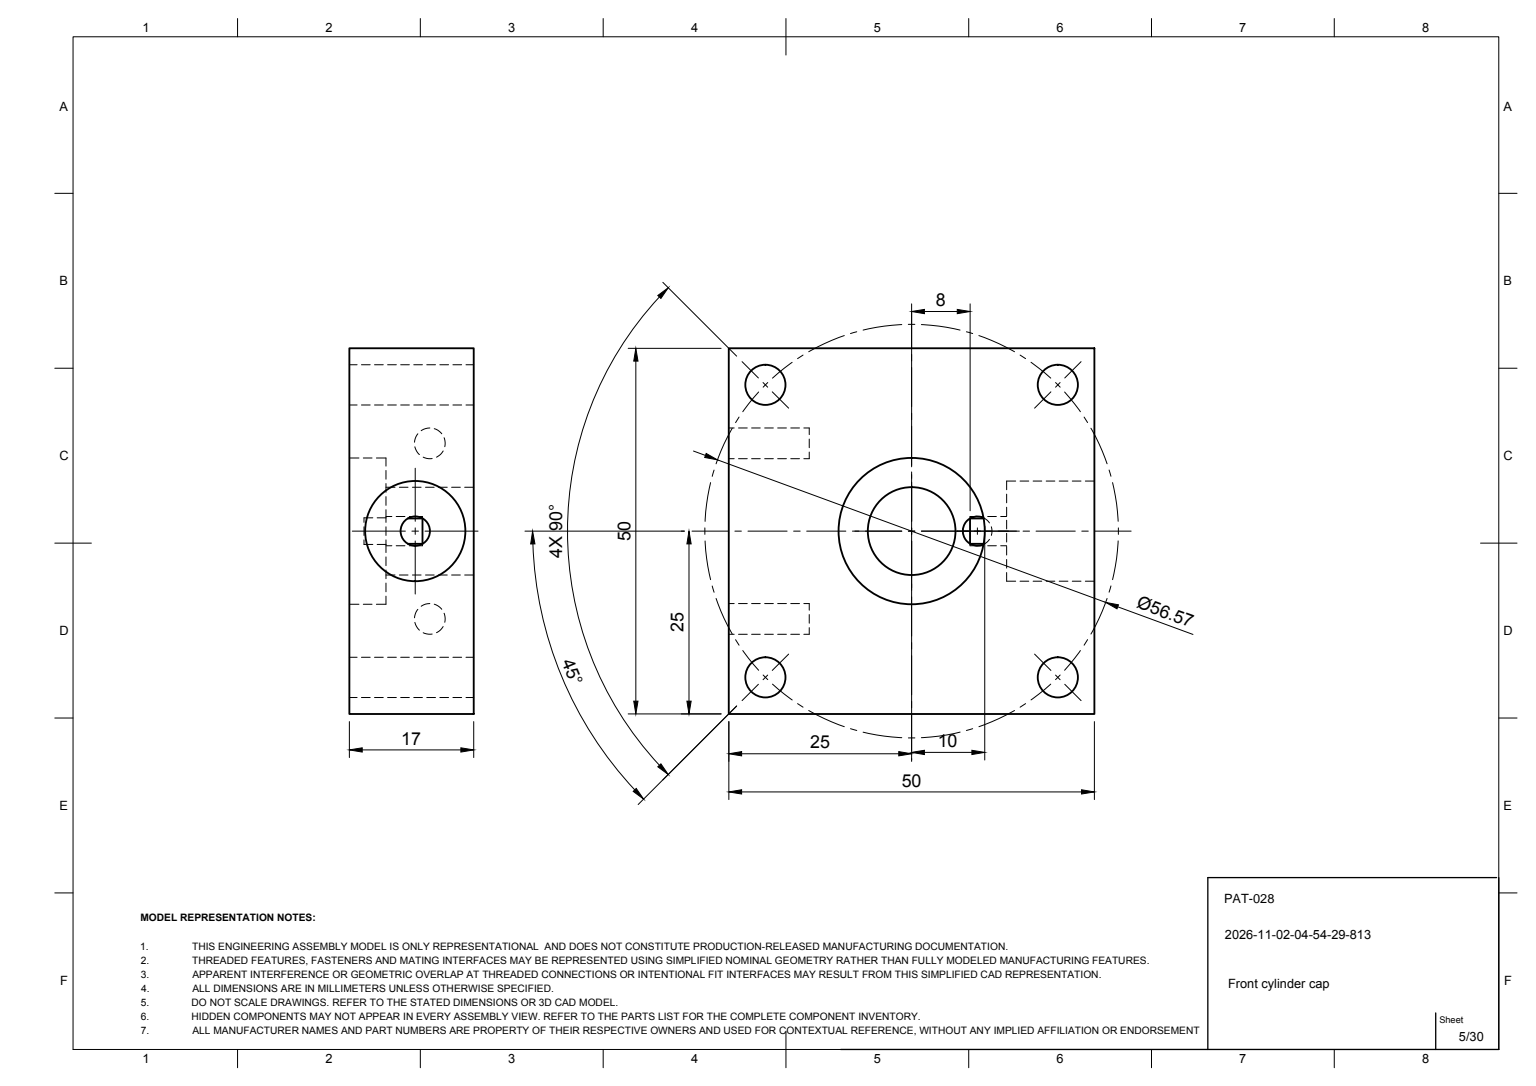
ISO-10303-21;
HEADER;
/* Generated by software containing ST-Developer
 * from STEP Tools, Inc. (www.steptools.com) 
 */

FILE_DESCRIPTION(
/* description */ ('Cylinder foot and clevis mount kit'),
/* implementation_level */ '2;1');

FILE_NAME(
/* name */ 'Front cylinder cap.step',
/* time_stamp */ '2026-10-27T20:10:43-07:00',
/* author */ (''),
/* organization */ (''),
/* preprocessor_version */ 'ST-DEVELOPER v20.2',
/* originating_system */ 'Autodesk Translation Framework v15.17.0.0',
/* authorisation */ '');

FILE_SCHEMA (('AUTOMOTIVE_DESIGN { 1 0 10303 214 3 1 1 }'));
ENDSEC;

DATA;
#10=MECHANICAL_DESIGN_GEOMETRIC_PRESENTATION_REPRESENTATION('',(#338),#9102);
#282=SHAPE_REPRESENTATION_RELATIONSHIP('SRR','None',#9229,#310);
#310=ADVANCED_BREP_SHAPE_REPRESENTATION('',(#366),#9072);
#338=STYLED_ITEM('',(#9446),#366);
#366=MANIFOLD_SOLID_BREP('Body1',#4924);
#392=FACE_BOUND('',#1021,.T.);
#393=FACE_BOUND('',#1028,.T.);
#394=FACE_BOUND('',#1030,.T.);
#395=FACE_BOUND('',#1031,.T.);
#396=FACE_BOUND('',#1032,.T.);
#397=FACE_BOUND('',#1033,.T.);
#398=FACE_BOUND('',#1034,.T.);
#399=FACE_BOUND('',#1037,.T.);
#400=FACE_BOUND('',#1038,.T.);
#401=FACE_BOUND('',#1039,.T.);
#402=FACE_BOUND('',#1040,.T.);
#403=FACE_BOUND('',#1041,.T.);
#404=FACE_BOUND('',#1044,.T.);
#405=FACE_BOUND('',#1046,.T.);
#406=FACE_BOUND('',#1047,.T.);
#495=ELLIPSE('',#5279,0.282842712474619,0.2);
#496=ELLIPSE('',#5280,0.282842712474619,0.2);
#497=ELLIPSE('',#5282,0.282842712474619,0.2);
#498=ELLIPSE('',#5283,0.282842712474619,0.2);
#499=ELLIPSE('',#5287,0.282842712474619,0.2);
#500=ELLIPSE('',#5289,0.282842712474619,0.2);
#501=ELLIPSE('',#5291,0.282842712474619,0.2);
#509=PLANE('',#5269);
#510=PLANE('',#5273);
#511=PLANE('',#5274);
#512=PLANE('',#5276);
#513=PLANE('',#5292);
#514=PLANE('',#5294);
#515=PLANE('',#5295);
#516=PLANE('',#5297);
#517=PLANE('',#5308);
#518=PLANE('',#5312);
#519=PLANE('',#5328);
#520=PLANE('',#5329);
#521=PLANE('',#5330);
#522=PLANE('',#5331);
#523=PLANE('',#5332);
#524=PLANE('',#5333);
#525=PLANE('',#5334);
#695=FACE_OUTER_BOUND('',#1001,.T.);
#696=FACE_OUTER_BOUND('',#1002,.T.);
#697=FACE_OUTER_BOUND('',#1003,.T.);
#698=FACE_OUTER_BOUND('',#1004,.T.);
#699=FACE_OUTER_BOUND('',#1005,.T.);
#700=FACE_OUTER_BOUND('',#1006,.T.);
#701=FACE_OUTER_BOUND('',#1007,.T.);
#702=FACE_OUTER_BOUND('',#1008,.T.);
#703=FACE_OUTER_BOUND('',#1009,.T.);
#704=FACE_OUTER_BOUND('',#1010,.T.);
#705=FACE_OUTER_BOUND('',#1011,.T.);
#706=FACE_OUTER_BOUND('',#1012,.T.);
#707=FACE_OUTER_BOUND('',#1013,.T.);
#708=FACE_OUTER_BOUND('',#1014,.T.);
#709=FACE_OUTER_BOUND('',#1015,.T.);
#710=FACE_OUTER_BOUND('',#1016,.T.);
#711=FACE_OUTER_BOUND('',#1017,.T.);
#712=FACE_OUTER_BOUND('',#1018,.T.);
#713=FACE_OUTER_BOUND('',#1019,.T.);
#714=FACE_OUTER_BOUND('',#1020,.T.);
#715=FACE_OUTER_BOUND('',#1022,.T.);
#716=FACE_OUTER_BOUND('',#1023,.T.);
#717=FACE_OUTER_BOUND('',#1024,.T.);
#718=FACE_OUTER_BOUND('',#1025,.T.);
#719=FACE_OUTER_BOUND('',#1026,.T.);
#720=FACE_OUTER_BOUND('',#1027,.T.);
#721=FACE_OUTER_BOUND('',#1029,.T.);
#722=FACE_OUTER_BOUND('',#1035,.T.);
#723=FACE_OUTER_BOUND('',#1036,.T.);
#724=FACE_OUTER_BOUND('',#1042,.T.);
#725=FACE_OUTER_BOUND('',#1043,.T.);
#726=FACE_OUTER_BOUND('',#1045,.T.);
#1001=EDGE_LOOP('',(#3315,#3316,#3317,#3318));
#1002=EDGE_LOOP('',(#3319));
#1003=EDGE_LOOP('',(#3320,#3321,#3322,#3323));
#1004=EDGE_LOOP('',(#3324));
#1005=EDGE_LOOP('',(#3325,#3326));
#1006=EDGE_LOOP('',(#3327,#3328));
#1007=EDGE_LOOP('',(#3329,#3330,#3331));
#1008=EDGE_LOOP('',(#3332,#3333,#3334,#3335,#3336,#3337,#3338,#3339,#3340,
#3341,#3342,#3343,#3344));
#1009=EDGE_LOOP('',(#3345,#3346,#3347));
#1010=EDGE_LOOP('',(#3348,#3349));
#1011=EDGE_LOOP('',(#3350,#3351));
#1012=EDGE_LOOP('',(#3352,#3353));
#1013=EDGE_LOOP('',(#3354,#3355));
#1014=EDGE_LOOP('',(#3356,#3357,#3358));
#1015=EDGE_LOOP('',(#3359,#3360,#3361,#3362,#3363,#3364,#3365,#3366,#3367));
#1016=EDGE_LOOP('',(#3368,#3369,#3370));
#1017=EDGE_LOOP('',(#3371,#3372,#3373,#3374,#3375,#3376,#3377,#3378));
#1018=EDGE_LOOP('',(#3379,#3380));
#1019=EDGE_LOOP('',(#3381,#3382,#3383,#3384));
#1020=EDGE_LOOP('',(#3385));
#1021=EDGE_LOOP('',(#3386));
#1022=EDGE_LOOP('',(#3387,#3388,#3389,#3390));
#1023=EDGE_LOOP('',(#3391,#3392,#3393,#3394));
#1024=EDGE_LOOP('',(#3395,#3396,#3397,#3398));
#1025=EDGE_LOOP('',(#3399,#3400,#3401,#3402));
#1026=EDGE_LOOP('',(#3403,#3404,#3405,#3406));
#1027=EDGE_LOOP('',(#3407,#3408,#3409,#3410));
#1028=EDGE_LOOP('',(#3411));
#1029=EDGE_LOOP('',(#3412,#3413,#3414,#3415));
#1030=EDGE_LOOP('',(#3416));
#1031=EDGE_LOOP('',(#3417));
#1032=EDGE_LOOP('',(#3418));
#1033=EDGE_LOOP('',(#3419));
#1034=EDGE_LOOP('',(#3420));
#1035=EDGE_LOOP('',(#3421,#3422,#3423,#3424));
#1036=EDGE_LOOP('',(#3425,#3426,#3427,#3428));
#1037=EDGE_LOOP('',(#3429));
#1038=EDGE_LOOP('',(#3430));
#1039=EDGE_LOOP('',(#3431));
#1040=EDGE_LOOP('',(#3432));
#1041=EDGE_LOOP('',(#3433));
#1042=EDGE_LOOP('',(#3434,#3435,#3436,#3437));
#1043=EDGE_LOOP('',(#3438,#3439,#3440,#3441));
#1044=EDGE_LOOP('',(#3442));
#1045=EDGE_LOOP('',(#3443,#3444,#3445,#3446));
#1046=EDGE_LOOP('',(#3447));
#1047=EDGE_LOOP('',(#3448));
#1410=LINE('',#7503,#1759);
#1411=LINE('',#7510,#1760);
#1412=LINE('',#7516,#1761);
#1413=LINE('',#7520,#1762);
#1414=LINE('',#7528,#1763);
#1415=LINE('',#7530,#1764);
#1416=LINE('',#7535,#1765);
#1417=LINE('',#7539,#1766);
#1418=LINE('',#7543,#1767);
#1419=LINE('',#7554,#1768);
#1420=LINE('',#7562,#1769);
#1421=LINE('',#7570,#1770);
#1422=LINE('',#7578,#1771);
#1423=LINE('',#7585,#1772);
#1424=LINE('',#7591,#1773);
#1425=LINE('',#7597,#1774);
#1426=LINE('',#7603,#1775);
#1427=LINE('',#7609,#1776);
#1428=LINE('',#7615,#1777);
#1429=LINE('',#7617,#1778);
#1430=LINE('',#7619,#1779);
#1431=LINE('',#7620,#1780);
#1432=LINE('',#7623,#1781);
#1433=LINE('',#7625,#1782);
#1434=LINE('',#7626,#1783);
#1435=LINE('',#7629,#1784);
#1436=LINE('',#7631,#1785);
#1437=LINE('',#7632,#1786);
#1438=LINE('',#7634,#1787);
#1439=LINE('',#7635,#1788);
#1759=VECTOR('',#5901,0.21);
#1760=VECTOR('',#5910,0.21);
#1761=VECTOR('',#5917,1.);
#1762=VECTOR('',#5922,1.);
#1763=VECTOR('',#5933,1.);
#1764=VECTOR('',#5934,1.);
#1765=VECTOR('',#5939,0.2);
#1766=VECTOR('',#5942,1.);
#1767=VECTOR('',#5945,1.);
#1768=VECTOR('',#5964,1.);
#1769=VECTOR('',#5977,0.2);
#1770=VECTOR('',#5988,1.);
#1771=VECTOR('',#5999,0.685);
#1772=VECTOR('',#6008,0.275);
#1773=VECTOR('',#6015,0.275);
#1774=VECTOR('',#6022,0.275);
#1775=VECTOR('',#6029,0.275);
#1776=VECTOR('',#6036,0.6);
#1777=VECTOR('',#6043,1.);
#1778=VECTOR('',#6044,1.);
#1779=VECTOR('',#6045,1.);
#1780=VECTOR('',#6046,1.);
#1781=VECTOR('',#6049,1.);
#1782=VECTOR('',#6050,1.);
#1783=VECTOR('',#6051,1.);
#1784=VECTOR('',#6054,1.);
#1785=VECTOR('',#6055,1.);
#1786=VECTOR('',#6056,1.);
#1787=VECTOR('',#6059,1.);
#1788=VECTOR('',#6060,1.);
#2108=CIRCLE('',#5267,0.21);
#2109=CIRCLE('',#5268,0.21);
#2110=CIRCLE('',#5271,0.21);
#2111=CIRCLE('',#5272,0.21);
#2112=CIRCLE('',#5275,0.2);
#2113=CIRCLE('',#5277,0.2);
#2114=CIRCLE('',#5284,0.2);
#2115=CIRCLE('',#5285,0.2);
#2116=CIRCLE('',#5286,0.2);
#2117=CIRCLE('',#5290,0.2);
#2118=CIRCLE('',#5293,1.);
#2119=CIRCLE('',#5296,0.2);
#2120=CIRCLE('',#5298,0.2);
#2121=CIRCLE('',#5301,0.2);
#2122=CIRCLE('',#5303,0.2);
#2123=CIRCLE('',#5305,1.);
#2124=CIRCLE('',#5306,1.);
#2125=CIRCLE('',#5307,1.);
#2126=CIRCLE('',#5310,0.685);
#2127=CIRCLE('',#5311,0.685);
#2128=CIRCLE('',#5314,0.275);
#2129=CIRCLE('',#5315,0.275);
#2130=CIRCLE('',#5317,0.275);
#2131=CIRCLE('',#5318,0.275);
#2132=CIRCLE('',#5320,0.275);
#2133=CIRCLE('',#5321,0.275);
#2134=CIRCLE('',#5323,0.275);
#2135=CIRCLE('',#5324,0.275);
#2136=CIRCLE('',#5326,0.6);
#2137=CIRCLE('',#5327,0.6);
#2328=VERTEX_POINT('',#7500);
#2329=VERTEX_POINT('',#7502);
#2330=VERTEX_POINT('',#7507);
#2331=VERTEX_POINT('',#7509);
#2332=VERTEX_POINT('',#7514);
#2333=VERTEX_POINT('',#7515);
#2334=VERTEX_POINT('',#7519);
#2335=VERTEX_POINT('',#7523);
#2336=VERTEX_POINT('',#7527);
#2337=VERTEX_POINT('',#7529);
#2338=VERTEX_POINT('',#7532);
#2339=VERTEX_POINT('',#7534);
#2340=VERTEX_POINT('',#7536);
#2341=VERTEX_POINT('',#7538);
#2342=VERTEX_POINT('',#7540);
#2343=VERTEX_POINT('',#7542);
#2344=VERTEX_POINT('',#7547);
#2345=VERTEX_POINT('',#7561);
#2346=VERTEX_POINT('',#7567);
#2347=VERTEX_POINT('',#7569);
#2348=VERTEX_POINT('',#7575);
#2349=VERTEX_POINT('',#7577);
#2350=VERTEX_POINT('',#7582);
#2351=VERTEX_POINT('',#7584);
#2352=VERTEX_POINT('',#7588);
#2353=VERTEX_POINT('',#7590);
#2354=VERTEX_POINT('',#7594);
#2355=VERTEX_POINT('',#7596);
#2356=VERTEX_POINT('',#7600);
#2357=VERTEX_POINT('',#7602);
#2358=VERTEX_POINT('',#7606);
#2359=VERTEX_POINT('',#7608);
#2360=VERTEX_POINT('',#7613);
#2361=VERTEX_POINT('',#7614);
#2362=VERTEX_POINT('',#7616);
#2363=VERTEX_POINT('',#7618);
#2364=VERTEX_POINT('',#7622);
#2365=VERTEX_POINT('',#7624);
#2366=VERTEX_POINT('',#7628);
#2367=VERTEX_POINT('',#7630);
#2712=EDGE_CURVE('',#2328,#2328,#2108,.T.);
#2713=EDGE_CURVE('',#2328,#2329,#1410,.T.);
#2714=EDGE_CURVE('',#2329,#2329,#2109,.T.);
#2715=EDGE_CURVE('',#2330,#2330,#2110,.T.);
#2716=EDGE_CURVE('',#2330,#2331,#1411,.T.);
#2717=EDGE_CURVE('',#2331,#2331,#2111,.T.);
#2718=EDGE_CURVE('',#2332,#2333,#1412,.T.);
#2719=EDGE_CURVE('',#2332,#2333,#2112,.T.);
#2720=EDGE_CURVE('',#2334,#2332,#1413,.T.);
#2721=EDGE_CURVE('',#2334,#2332,#2113,.T.);
#2722=EDGE_CURVE('',#2335,#2334,#495,.T.);
#2723=EDGE_CURVE('',#2332,#2335,#496,.T.);
#2724=EDGE_CURVE('',#2333,#2336,#1414,.T.);
#2725=EDGE_CURVE('',#2337,#2332,#1415,.T.);
#2726=EDGE_CURVE('',#2335,#2337,#497,.T.);
#2727=EDGE_CURVE('',#2338,#2335,#498,.T.);
#2728=EDGE_CURVE('',#2338,#2339,#1416,.T.);
#2729=EDGE_CURVE('',#2340,#2339,#2114,.T.);
#2730=EDGE_CURVE('',#2341,#2340,#1417,.T.);
#2731=EDGE_CURVE('',#2341,#2342,#2115,.T.);
#2732=EDGE_CURVE('',#2343,#2342,#1418,.T.);
#2733=EDGE_CURVE('',#2339,#2343,#2116,.T.);
#2734=EDGE_CURVE('',#2336,#2338,#499,.T.);
#2735=EDGE_CURVE('',#2344,#2338,#500,.T.);
#2736=EDGE_CURVE('',#2333,#2344,#2117,.T.);
#2737=EDGE_CURVE('',#2338,#2333,#501,.T.);
#2738=EDGE_CURVE('',#2342,#2341,#2118,.T.);
#2739=EDGE_CURVE('',#2333,#2344,#1419,.T.);
#2740=EDGE_CURVE('',#2332,#2337,#2119,.T.);
#2741=EDGE_CURVE('',#2333,#2332,#2120,.T.);
#2742=EDGE_CURVE('',#2338,#2345,#1420,.T.);
#2743=EDGE_CURVE('',#2345,#2345,#2121,.T.);
#2744=EDGE_CURVE('',#2336,#2333,#2122,.T.);
#2745=EDGE_CURVE('',#2346,#2340,#2123,.T.);
#2746=EDGE_CURVE('',#2346,#2347,#1421,.T.);
#2747=EDGE_CURVE('',#2347,#2347,#2124,.T.);
#2748=EDGE_CURVE('',#2343,#2346,#2125,.T.);
#2749=EDGE_CURVE('',#2348,#2348,#2126,.T.);
#2750=EDGE_CURVE('',#2348,#2349,#1422,.T.);
#2751=EDGE_CURVE('',#2349,#2349,#2127,.T.);
#2752=EDGE_CURVE('',#2350,#2350,#2128,.T.);
#2753=EDGE_CURVE('',#2350,#2351,#1423,.T.);
#2754=EDGE_CURVE('',#2351,#2351,#2129,.T.);
#2755=EDGE_CURVE('',#2352,#2352,#2130,.T.);
#2756=EDGE_CURVE('',#2352,#2353,#1424,.T.);
#2757=EDGE_CURVE('',#2353,#2353,#2131,.T.);
#2758=EDGE_CURVE('',#2354,#2354,#2132,.T.);
#2759=EDGE_CURVE('',#2354,#2355,#1425,.T.);
#2760=EDGE_CURVE('',#2355,#2355,#2133,.T.);
#2761=EDGE_CURVE('',#2356,#2356,#2134,.T.);
#2762=EDGE_CURVE('',#2356,#2357,#1426,.T.);
#2763=EDGE_CURVE('',#2357,#2357,#2135,.T.);
#2764=EDGE_CURVE('',#2358,#2358,#2136,.T.);
#2765=EDGE_CURVE('',#2358,#2359,#1427,.T.);
#2766=EDGE_CURVE('',#2359,#2359,#2137,.T.);
#2767=EDGE_CURVE('',#2360,#2361,#1428,.T.);
#2768=EDGE_CURVE('',#2361,#2362,#1429,.T.);
#2769=EDGE_CURVE('',#2363,#2362,#1430,.T.);
#2770=EDGE_CURVE('',#2360,#2363,#1431,.T.);
#2771=EDGE_CURVE('',#2364,#2360,#1432,.T.);
#2772=EDGE_CURVE('',#2365,#2363,#1433,.T.);
#2773=EDGE_CURVE('',#2364,#2365,#1434,.T.);
#2774=EDGE_CURVE('',#2366,#2364,#1435,.T.);
#2775=EDGE_CURVE('',#2367,#2365,#1436,.T.);
#2776=EDGE_CURVE('',#2366,#2367,#1437,.T.);
#2777=EDGE_CURVE('',#2361,#2366,#1438,.T.);
#2778=EDGE_CURVE('',#2362,#2367,#1439,.T.);
#3315=ORIENTED_EDGE('',*,*,#2712,.F.);
#3316=ORIENTED_EDGE('',*,*,#2713,.T.);
#3317=ORIENTED_EDGE('',*,*,#2714,.T.);
#3318=ORIENTED_EDGE('',*,*,#2713,.F.);
#3319=ORIENTED_EDGE('',*,*,#2714,.F.);
#3320=ORIENTED_EDGE('',*,*,#2715,.F.);
#3321=ORIENTED_EDGE('',*,*,#2716,.T.);
#3322=ORIENTED_EDGE('',*,*,#2717,.T.);
#3323=ORIENTED_EDGE('',*,*,#2716,.F.);
#3324=ORIENTED_EDGE('',*,*,#2717,.F.);
#3325=ORIENTED_EDGE('',*,*,#2718,.F.);
#3326=ORIENTED_EDGE('',*,*,#2719,.T.);
#3327=ORIENTED_EDGE('',*,*,#2720,.F.);
#3328=ORIENTED_EDGE('',*,*,#2721,.T.);
#3329=ORIENTED_EDGE('',*,*,#2722,.F.);
#3330=ORIENTED_EDGE('',*,*,#2723,.F.);
#3331=ORIENTED_EDGE('',*,*,#2721,.F.);
#3332=ORIENTED_EDGE('',*,*,#2724,.F.);
#3333=ORIENTED_EDGE('',*,*,#2719,.F.);
#3334=ORIENTED_EDGE('',*,*,#2725,.F.);
#3335=ORIENTED_EDGE('',*,*,#2726,.F.);
#3336=ORIENTED_EDGE('',*,*,#2727,.F.);
#3337=ORIENTED_EDGE('',*,*,#2728,.T.);
#3338=ORIENTED_EDGE('',*,*,#2729,.F.);
#3339=ORIENTED_EDGE('',*,*,#2730,.F.);
#3340=ORIENTED_EDGE('',*,*,#2731,.T.);
#3341=ORIENTED_EDGE('',*,*,#2732,.F.);
#3342=ORIENTED_EDGE('',*,*,#2733,.F.);
#3343=ORIENTED_EDGE('',*,*,#2728,.F.);
#3344=ORIENTED_EDGE('',*,*,#2734,.F.);
#3345=ORIENTED_EDGE('',*,*,#2735,.F.);
#3346=ORIENTED_EDGE('',*,*,#2736,.F.);
#3347=ORIENTED_EDGE('',*,*,#2737,.F.);
#3348=ORIENTED_EDGE('',*,*,#2738,.F.);
#3349=ORIENTED_EDGE('',*,*,#2731,.F.);
#3350=ORIENTED_EDGE('',*,*,#2739,.F.);
#3351=ORIENTED_EDGE('',*,*,#2736,.T.);
#3352=ORIENTED_EDGE('',*,*,#2725,.T.);
#3353=ORIENTED_EDGE('',*,*,#2740,.T.);
#3354=ORIENTED_EDGE('',*,*,#2718,.T.);
#3355=ORIENTED_EDGE('',*,*,#2741,.T.);
#3356=ORIENTED_EDGE('',*,*,#2726,.T.);
#3357=ORIENTED_EDGE('',*,*,#2740,.F.);
#3358=ORIENTED_EDGE('',*,*,#2723,.T.);
#3359=ORIENTED_EDGE('',*,*,#2739,.T.);
#3360=ORIENTED_EDGE('',*,*,#2735,.T.);
#3361=ORIENTED_EDGE('',*,*,#2742,.T.);
#3362=ORIENTED_EDGE('',*,*,#2743,.F.);
#3363=ORIENTED_EDGE('',*,*,#2742,.F.);
#3364=ORIENTED_EDGE('',*,*,#2727,.T.);
#3365=ORIENTED_EDGE('',*,*,#2722,.T.);
#3366=ORIENTED_EDGE('',*,*,#2720,.T.);
#3367=ORIENTED_EDGE('',*,*,#2741,.F.);
#3368=ORIENTED_EDGE('',*,*,#2734,.T.);
#3369=ORIENTED_EDGE('',*,*,#2737,.T.);
#3370=ORIENTED_EDGE('',*,*,#2744,.F.);
#3371=ORIENTED_EDGE('',*,*,#2732,.T.);
#3372=ORIENTED_EDGE('',*,*,#2738,.T.);
#3373=ORIENTED_EDGE('',*,*,#2730,.T.);
#3374=ORIENTED_EDGE('',*,*,#2745,.F.);
#3375=ORIENTED_EDGE('',*,*,#2746,.T.);
#3376=ORIENTED_EDGE('',*,*,#2747,.F.);
#3377=ORIENTED_EDGE('',*,*,#2746,.F.);
#3378=ORIENTED_EDGE('',*,*,#2748,.F.);
#3379=ORIENTED_EDGE('',*,*,#2724,.T.);
#3380=ORIENTED_EDGE('',*,*,#2744,.T.);
#3381=ORIENTED_EDGE('',*,*,#2749,.F.);
#3382=ORIENTED_EDGE('',*,*,#2750,.T.);
#3383=ORIENTED_EDGE('',*,*,#2751,.F.);
#3384=ORIENTED_EDGE('',*,*,#2750,.F.);
#3385=ORIENTED_EDGE('',*,*,#2749,.T.);
#3386=ORIENTED_EDGE('',*,*,#2743,.T.);
#3387=ORIENTED_EDGE('',*,*,#2752,.F.);
#3388=ORIENTED_EDGE('',*,*,#2753,.T.);
#3389=ORIENTED_EDGE('',*,*,#2754,.F.);
#3390=ORIENTED_EDGE('',*,*,#2753,.F.);
#3391=ORIENTED_EDGE('',*,*,#2755,.F.);
#3392=ORIENTED_EDGE('',*,*,#2756,.T.);
#3393=ORIENTED_EDGE('',*,*,#2757,.F.);
#3394=ORIENTED_EDGE('',*,*,#2756,.F.);
#3395=ORIENTED_EDGE('',*,*,#2758,.F.);
#3396=ORIENTED_EDGE('',*,*,#2759,.T.);
#3397=ORIENTED_EDGE('',*,*,#2760,.F.);
#3398=ORIENTED_EDGE('',*,*,#2759,.F.);
#3399=ORIENTED_EDGE('',*,*,#2761,.F.);
#3400=ORIENTED_EDGE('',*,*,#2762,.T.);
#3401=ORIENTED_EDGE('',*,*,#2763,.F.);
#3402=ORIENTED_EDGE('',*,*,#2762,.F.);
#3403=ORIENTED_EDGE('',*,*,#2764,.F.);
#3404=ORIENTED_EDGE('',*,*,#2765,.T.);
#3405=ORIENTED_EDGE('',*,*,#2766,.F.);
#3406=ORIENTED_EDGE('',*,*,#2765,.F.);
#3407=ORIENTED_EDGE('',*,*,#2729,.T.);
#3408=ORIENTED_EDGE('',*,*,#2733,.T.);
#3409=ORIENTED_EDGE('',*,*,#2748,.T.);
#3410=ORIENTED_EDGE('',*,*,#2745,.T.);
#3411=ORIENTED_EDGE('',*,*,#2766,.T.);
#3412=ORIENTED_EDGE('',*,*,#2767,.T.);
#3413=ORIENTED_EDGE('',*,*,#2768,.T.);
#3414=ORIENTED_EDGE('',*,*,#2769,.F.);
#3415=ORIENTED_EDGE('',*,*,#2770,.F.);
#3416=ORIENTED_EDGE('',*,*,#2747,.T.);
#3417=ORIENTED_EDGE('',*,*,#2763,.T.);
#3418=ORIENTED_EDGE('',*,*,#2760,.T.);
#3419=ORIENTED_EDGE('',*,*,#2757,.T.);
#3420=ORIENTED_EDGE('',*,*,#2754,.T.);
#3421=ORIENTED_EDGE('',*,*,#2771,.T.);
#3422=ORIENTED_EDGE('',*,*,#2770,.T.);
#3423=ORIENTED_EDGE('',*,*,#2772,.F.);
#3424=ORIENTED_EDGE('',*,*,#2773,.F.);
#3425=ORIENTED_EDGE('',*,*,#2774,.T.);
#3426=ORIENTED_EDGE('',*,*,#2773,.T.);
#3427=ORIENTED_EDGE('',*,*,#2775,.F.);
#3428=ORIENTED_EDGE('',*,*,#2776,.F.);
#3429=ORIENTED_EDGE('',*,*,#2764,.T.);
#3430=ORIENTED_EDGE('',*,*,#2761,.T.);
#3431=ORIENTED_EDGE('',*,*,#2758,.T.);
#3432=ORIENTED_EDGE('',*,*,#2755,.T.);
#3433=ORIENTED_EDGE('',*,*,#2752,.T.);
#3434=ORIENTED_EDGE('',*,*,#2777,.T.);
#3435=ORIENTED_EDGE('',*,*,#2776,.T.);
#3436=ORIENTED_EDGE('',*,*,#2778,.F.);
#3437=ORIENTED_EDGE('',*,*,#2768,.F.);
#3438=ORIENTED_EDGE('',*,*,#2778,.T.);
#3439=ORIENTED_EDGE('',*,*,#2775,.T.);
#3440=ORIENTED_EDGE('',*,*,#2772,.T.);
#3441=ORIENTED_EDGE('',*,*,#2769,.T.);
#3442=ORIENTED_EDGE('',*,*,#2751,.T.);
#3443=ORIENTED_EDGE('',*,*,#2777,.F.);
#3444=ORIENTED_EDGE('',*,*,#2767,.F.);
#3445=ORIENTED_EDGE('',*,*,#2771,.F.);
#3446=ORIENTED_EDGE('',*,*,#2774,.F.);
#3447=ORIENTED_EDGE('',*,*,#2712,.T.);
#3448=ORIENTED_EDGE('',*,*,#2715,.T.);
#4521=CYLINDRICAL_SURFACE('',#5266,0.21);
#4522=CYLINDRICAL_SURFACE('',#5270,0.21);
#4523=CYLINDRICAL_SURFACE('',#5278,0.2);
#4524=CYLINDRICAL_SURFACE('',#5281,0.2);
#4525=CYLINDRICAL_SURFACE('',#5288,0.2);
#4526=CYLINDRICAL_SURFACE('',#5299,0.2);
#4527=CYLINDRICAL_SURFACE('',#5300,0.2);
#4528=CYLINDRICAL_SURFACE('',#5302,0.2);
#4529=CYLINDRICAL_SURFACE('',#5304,1.);
#4530=CYLINDRICAL_SURFACE('',#5309,0.685);
#4531=CYLINDRICAL_SURFACE('',#5313,0.275);
#4532=CYLINDRICAL_SURFACE('',#5316,0.275);
#4533=CYLINDRICAL_SURFACE('',#5319,0.275);
#4534=CYLINDRICAL_SURFACE('',#5322,0.275);
#4535=CYLINDRICAL_SURFACE('',#5325,0.6);
#4618=ADVANCED_FACE('',(#695),#4521,.F.);
#4619=ADVANCED_FACE('',(#696),#509,.F.);
#4620=ADVANCED_FACE('',(#697),#4522,.F.);
#4621=ADVANCED_FACE('',(#698),#510,.F.);
#4622=ADVANCED_FACE('',(#699),#511,.T.);
#4623=ADVANCED_FACE('',(#700),#512,.T.);
#4624=ADVANCED_FACE('',(#701),#4523,.F.);
#4625=ADVANCED_FACE('',(#702),#4524,.F.);
#4626=ADVANCED_FACE('',(#703),#4525,.F.);
#4627=ADVANCED_FACE('',(#704),#513,.F.);
#4628=ADVANCED_FACE('',(#705),#514,.T.);
#4629=ADVANCED_FACE('',(#706),#515,.T.);
#4630=ADVANCED_FACE('',(#707),#516,.T.);
#4631=ADVANCED_FACE('',(#708),#4526,.F.);
#4632=ADVANCED_FACE('',(#709),#4527,.F.);
#4633=ADVANCED_FACE('',(#710),#4528,.F.);
#4634=ADVANCED_FACE('',(#711),#4529,.F.);
#4635=ADVANCED_FACE('',(#712),#517,.T.);
#4636=ADVANCED_FACE('',(#713),#4530,.F.);
#4637=ADVANCED_FACE('',(#714,#392),#518,.T.);
#4638=ADVANCED_FACE('',(#715),#4531,.F.);
#4639=ADVANCED_FACE('',(#716),#4532,.F.);
#4640=ADVANCED_FACE('',(#717),#4533,.F.);
#4641=ADVANCED_FACE('',(#718),#4534,.F.);
#4642=ADVANCED_FACE('',(#719),#4535,.F.);
#4643=ADVANCED_FACE('',(#720,#393),#519,.T.);
#4644=ADVANCED_FACE('',(#721,#394,#395,#396,#397,#398),#520,.T.);
#4645=ADVANCED_FACE('',(#722),#521,.T.);
#4646=ADVANCED_FACE('',(#723,#399,#400,#401,#402,#403),#522,.T.);
#4647=ADVANCED_FACE('',(#724),#523,.T.);
#4648=ADVANCED_FACE('',(#725,#404),#524,.T.);
#4649=ADVANCED_FACE('',(#726,#405,#406),#525,.F.);
#4924=CLOSED_SHELL('',(#4618,#4619,#4620,#4621,#4622,#4623,#4624,#4625,
#4626,#4627,#4628,#4629,#4630,#4631,#4632,#4633,#4634,#4635,#4636,#4637,
#4638,#4639,#4640,#4641,#4642,#4643,#4644,#4645,#4646,#4647,#4648,#4649));
#5265=AXIS2_PLACEMENT_3D('',#7498,#5895,#5896);
#5266=AXIS2_PLACEMENT_3D('',#7499,#5897,#5898);
#5267=AXIS2_PLACEMENT_3D('',#7501,#5899,#5900);
#5268=AXIS2_PLACEMENT_3D('',#7504,#5902,#5903);
#5269=AXIS2_PLACEMENT_3D('',#7505,#5904,#5905);
#5270=AXIS2_PLACEMENT_3D('',#7506,#5906,#5907);
#5271=AXIS2_PLACEMENT_3D('',#7508,#5908,#5909);
#5272=AXIS2_PLACEMENT_3D('',#7511,#5911,#5912);
#5273=AXIS2_PLACEMENT_3D('',#7512,#5913,#5914);
#5274=AXIS2_PLACEMENT_3D('',#7513,#5915,#5916);
#5275=AXIS2_PLACEMENT_3D('',#7517,#5918,#5919);
#5276=AXIS2_PLACEMENT_3D('',#7518,#5920,#5921);
#5277=AXIS2_PLACEMENT_3D('',#7521,#5923,#5924);
#5278=AXIS2_PLACEMENT_3D('',#7522,#5925,#5926);
#5279=AXIS2_PLACEMENT_3D('',#7524,#5927,#5928);
#5280=AXIS2_PLACEMENT_3D('',#7525,#5929,#5930);
#5281=AXIS2_PLACEMENT_3D('',#7526,#5931,#5932);
#5282=AXIS2_PLACEMENT_3D('',#7531,#5935,#5936);
#5283=AXIS2_PLACEMENT_3D('',#7533,#5937,#5938);
#5284=AXIS2_PLACEMENT_3D('',#7537,#5940,#5941);
#5285=AXIS2_PLACEMENT_3D('',#7541,#5943,#5944);
#5286=AXIS2_PLACEMENT_3D('',#7544,#5946,#5947);
#5287=AXIS2_PLACEMENT_3D('',#7545,#5948,#5949);
#5288=AXIS2_PLACEMENT_3D('',#7546,#5950,#5951);
#5289=AXIS2_PLACEMENT_3D('',#7548,#5952,#5953);
#5290=AXIS2_PLACEMENT_3D('',#7549,#5954,#5955);
#5291=AXIS2_PLACEMENT_3D('',#7550,#5956,#5957);
#5292=AXIS2_PLACEMENT_3D('',#7551,#5958,#5959);
#5293=AXIS2_PLACEMENT_3D('',#7552,#5960,#5961);
#5294=AXIS2_PLACEMENT_3D('',#7553,#5962,#5963);
#5295=AXIS2_PLACEMENT_3D('',#7555,#5965,#5966);
#5296=AXIS2_PLACEMENT_3D('',#7556,#5967,#5968);
#5297=AXIS2_PLACEMENT_3D('',#7557,#5969,#5970);
#5298=AXIS2_PLACEMENT_3D('',#7558,#5971,#5972);
#5299=AXIS2_PLACEMENT_3D('',#7559,#5973,#5974);
#5300=AXIS2_PLACEMENT_3D('',#7560,#5975,#5976);
#5301=AXIS2_PLACEMENT_3D('',#7563,#5978,#5979);
#5302=AXIS2_PLACEMENT_3D('',#7564,#5980,#5981);
#5303=AXIS2_PLACEMENT_3D('',#7565,#5982,#5983);
#5304=AXIS2_PLACEMENT_3D('',#7566,#5984,#5985);
#5305=AXIS2_PLACEMENT_3D('',#7568,#5986,#5987);
#5306=AXIS2_PLACEMENT_3D('',#7571,#5989,#5990);
#5307=AXIS2_PLACEMENT_3D('',#7572,#5991,#5992);
#5308=AXIS2_PLACEMENT_3D('',#7573,#5993,#5994);
#5309=AXIS2_PLACEMENT_3D('',#7574,#5995,#5996);
#5310=AXIS2_PLACEMENT_3D('',#7576,#5997,#5998);
#5311=AXIS2_PLACEMENT_3D('',#7579,#6000,#6001);
#5312=AXIS2_PLACEMENT_3D('',#7580,#6002,#6003);
#5313=AXIS2_PLACEMENT_3D('',#7581,#6004,#6005);
#5314=AXIS2_PLACEMENT_3D('',#7583,#6006,#6007);
#5315=AXIS2_PLACEMENT_3D('',#7586,#6009,#6010);
#5316=AXIS2_PLACEMENT_3D('',#7587,#6011,#6012);
#5317=AXIS2_PLACEMENT_3D('',#7589,#6013,#6014);
#5318=AXIS2_PLACEMENT_3D('',#7592,#6016,#6017);
#5319=AXIS2_PLACEMENT_3D('',#7593,#6018,#6019);
#5320=AXIS2_PLACEMENT_3D('',#7595,#6020,#6021);
#5321=AXIS2_PLACEMENT_3D('',#7598,#6023,#6024);
#5322=AXIS2_PLACEMENT_3D('',#7599,#6025,#6026);
#5323=AXIS2_PLACEMENT_3D('',#7601,#6027,#6028);
#5324=AXIS2_PLACEMENT_3D('',#7604,#6030,#6031);
#5325=AXIS2_PLACEMENT_3D('',#7605,#6032,#6033);
#5326=AXIS2_PLACEMENT_3D('',#7607,#6034,#6035);
#5327=AXIS2_PLACEMENT_3D('',#7610,#6037,#6038);
#5328=AXIS2_PLACEMENT_3D('',#7611,#6039,#6040);
#5329=AXIS2_PLACEMENT_3D('',#7612,#6041,#6042);
#5330=AXIS2_PLACEMENT_3D('',#7621,#6047,#6048);
#5331=AXIS2_PLACEMENT_3D('',#7627,#6052,#6053);
#5332=AXIS2_PLACEMENT_3D('',#7633,#6057,#6058);
#5333=AXIS2_PLACEMENT_3D('',#7636,#6061,#6062);
#5334=AXIS2_PLACEMENT_3D('',#7637,#6063,#6064);
#5895=DIRECTION('axis',(0.,0.,1.));
#5896=DIRECTION('refdir',(1.,0.,0.));
#5897=DIRECTION('center_axis',(0.,0.,1.));
#5898=DIRECTION('ref_axis',(1.,0.,0.));
#5899=DIRECTION('center_axis',(0.,0.,1.));
#5900=DIRECTION('ref_axis',(1.,0.,0.));
#5901=DIRECTION('',(0.,0.,1.));
#5902=DIRECTION('center_axis',(0.,0.,1.));
#5903=DIRECTION('ref_axis',(1.,0.,0.));
#5904=DIRECTION('center_axis',(0.,0.,1.));
#5905=DIRECTION('ref_axis',(1.,0.,0.));
#5906=DIRECTION('center_axis',(0.,0.,1.));
#5907=DIRECTION('ref_axis',(1.,0.,0.));
#5908=DIRECTION('center_axis',(0.,0.,1.));
#5909=DIRECTION('ref_axis',(1.,0.,0.));
#5910=DIRECTION('',(0.,0.,1.));
#5911=DIRECTION('center_axis',(0.,0.,1.));
#5912=DIRECTION('ref_axis',(1.,0.,0.));
#5913=DIRECTION('center_axis',(0.,0.,1.));
#5914=DIRECTION('ref_axis',(1.,0.,0.));
#5915=DIRECTION('center_axis',(0.,1.,0.));
#5916=DIRECTION('ref_axis',(1.,0.,0.));
#5917=DIRECTION('',(-1.,0.,0.));
#5918=DIRECTION('center_axis',(0.,1.,0.));
#5919=DIRECTION('ref_axis',(1.,0.,0.));
#5920=DIRECTION('center_axis',(0.,1.,0.));
#5921=DIRECTION('ref_axis',(1.,0.,0.));
#5922=DIRECTION('',(0.,0.,-1.));
#5923=DIRECTION('center_axis',(0.,1.,0.));
#5924=DIRECTION('ref_axis',(1.,0.,0.));
#5925=DIRECTION('center_axis',(0.,1.,0.));
#5926=DIRECTION('ref_axis',(1.,0.,0.));
#5927=DIRECTION('center_axis',(0.,-0.707106781186548,-0.707106781186547));
#5928=DIRECTION('ref_axis',(0.,0.707106781186547,-0.707106781186548));
#5929=DIRECTION('center_axis',(0.,-0.707106781186548,0.707106781186547));
#5930=DIRECTION('ref_axis',(0.,-0.707106781186547,-0.707106781186548));
#5931=DIRECTION('center_axis',(0.,1.,0.));
#5932=DIRECTION('ref_axis',(1.,0.,0.));
#5933=DIRECTION('',(0.,1.,0.));
#5934=DIRECTION('',(0.,-1.,0.));
#5935=DIRECTION('center_axis',(0.,0.707106781186548,0.707106781186547));
#5936=DIRECTION('ref_axis',(0.,0.707106781186547,-0.707106781186548));
#5937=DIRECTION('center_axis',(0.,0.707106781186548,-0.707106781186547));
#5938=DIRECTION('ref_axis',(0.,-0.707106781186547,-0.707106781186548));
#5939=DIRECTION('',(0.,1.,0.));
#5940=DIRECTION('center_axis',(0.,-1.,0.));
#5941=DIRECTION('ref_axis',(1.,0.,0.));
#5942=DIRECTION('',(0.,-1.,0.));
#5943=DIRECTION('center_axis',(0.,1.,0.));
#5944=DIRECTION('ref_axis',(1.,0.,0.));
#5945=DIRECTION('',(0.,1.,0.));
#5946=DIRECTION('center_axis',(0.,-1.,0.));
#5947=DIRECTION('ref_axis',(1.,0.,0.));
#5948=DIRECTION('center_axis',(0.,0.707106781186548,0.707106781186547));
#5949=DIRECTION('ref_axis',(0.,0.707106781186547,-0.707106781186548));
#5950=DIRECTION('center_axis',(0.,1.,0.));
#5951=DIRECTION('ref_axis',(-1.,0.,-2.54207057918564E-15));
#5952=DIRECTION('center_axis',(0.,-0.707106781186548,-0.707106781186547));
#5953=DIRECTION('ref_axis',(0.,0.707106781186547,-0.707106781186548));
#5954=DIRECTION('center_axis',(0.,1.,0.));
#5955=DIRECTION('ref_axis',(1.,0.,0.));
#5956=DIRECTION('center_axis',(0.,-0.707106781186548,0.707106781186547));
#5957=DIRECTION('ref_axis',(0.,-0.707106781186547,-0.707106781186548));
#5958=DIRECTION('center_axis',(0.,1.,0.));
#5959=DIRECTION('ref_axis',(1.,0.,0.));
#5960=DIRECTION('center_axis',(0.,-1.,0.));
#5961=DIRECTION('ref_axis',(1.,0.,0.));
#5962=DIRECTION('center_axis',(0.,1.,0.));
#5963=DIRECTION('ref_axis',(1.,0.,0.));
#5964=DIRECTION('',(0.,0.,1.));
#5965=DIRECTION('center_axis',(0.,0.,1.));
#5966=DIRECTION('ref_axis',(1.,0.,0.));
#5967=DIRECTION('center_axis',(0.,0.,1.));
#5968=DIRECTION('ref_axis',(1.,0.,0.));
#5969=DIRECTION('center_axis',(0.,0.,1.));
#5970=DIRECTION('ref_axis',(1.,0.,0.));
#5971=DIRECTION('center_axis',(0.,0.,1.));
#5972=DIRECTION('ref_axis',(1.,0.,0.));
#5973=DIRECTION('center_axis',(0.,0.,1.));
#5974=DIRECTION('ref_axis',(1.,0.,0.));
#5975=DIRECTION('center_axis',(0.,0.,1.));
#5976=DIRECTION('ref_axis',(1.,0.,0.));
#5977=DIRECTION('',(0.,0.,1.));
#5978=DIRECTION('center_axis',(0.,0.,-1.));
#5979=DIRECTION('ref_axis',(1.,0.,0.));
#5980=DIRECTION('center_axis',(0.,0.,1.));
#5981=DIRECTION('ref_axis',(-1.,-1.65389215948552E-15,0.));
#5982=DIRECTION('center_axis',(0.,0.,1.));
#5983=DIRECTION('ref_axis',(1.,0.,0.));
#5984=DIRECTION('center_axis',(0.,1.,0.));
#5985=DIRECTION('ref_axis',(1.,0.,0.));
#5986=DIRECTION('center_axis',(0.,1.,0.));
#5987=DIRECTION('ref_axis',(1.,0.,0.));
#5988=DIRECTION('',(0.,1.,0.));
#5989=DIRECTION('center_axis',(0.,-1.,0.));
#5990=DIRECTION('ref_axis',(1.,0.,0.));
#5991=DIRECTION('center_axis',(0.,1.,0.));
#5992=DIRECTION('ref_axis',(1.,0.,0.));
#5993=DIRECTION('center_axis',(0.,0.,1.));
#5994=DIRECTION('ref_axis',(1.,0.,0.));
#5995=DIRECTION('center_axis',(0.,0.,1.));
#5996=DIRECTION('ref_axis',(1.,0.,0.));
#5997=DIRECTION('center_axis',(0.,0.,1.));
#5998=DIRECTION('ref_axis',(1.,0.,0.));
#5999=DIRECTION('',(0.,0.,1.));
#6000=DIRECTION('center_axis',(0.,0.,-1.));
#6001=DIRECTION('ref_axis',(1.,0.,0.));
#6002=DIRECTION('center_axis',(0.,0.,1.));
#6003=DIRECTION('ref_axis',(1.,0.,0.));
#6004=DIRECTION('center_axis',(0.,1.,0.));
#6005=DIRECTION('ref_axis',(1.,0.,0.));
#6006=DIRECTION('center_axis',(0.,1.,0.));
#6007=DIRECTION('ref_axis',(1.,0.,0.));
#6008=DIRECTION('',(0.,1.,0.));
#6009=DIRECTION('center_axis',(0.,-1.,0.));
#6010=DIRECTION('ref_axis',(1.,0.,0.));
#6011=DIRECTION('center_axis',(0.,1.,0.));
#6012=DIRECTION('ref_axis',(1.,0.,0.));
#6013=DIRECTION('center_axis',(0.,1.,0.));
#6014=DIRECTION('ref_axis',(1.,0.,0.));
#6015=DIRECTION('',(0.,1.,0.));
#6016=DIRECTION('center_axis',(0.,-1.,0.));
#6017=DIRECTION('ref_axis',(1.,0.,0.));
#6018=DIRECTION('center_axis',(0.,1.,0.));
#6019=DIRECTION('ref_axis',(1.,0.,0.));
#6020=DIRECTION('center_axis',(0.,1.,0.));
#6021=DIRECTION('ref_axis',(1.,0.,0.));
#6022=DIRECTION('',(0.,1.,0.));
#6023=DIRECTION('center_axis',(0.,-1.,0.));
#6024=DIRECTION('ref_axis',(1.,0.,0.));
#6025=DIRECTION('center_axis',(0.,1.,0.));
#6026=DIRECTION('ref_axis',(1.,0.,0.));
#6027=DIRECTION('center_axis',(0.,1.,0.));
#6028=DIRECTION('ref_axis',(1.,0.,0.));
#6029=DIRECTION('',(0.,1.,0.));
#6030=DIRECTION('center_axis',(0.,-1.,0.));
#6031=DIRECTION('ref_axis',(1.,0.,0.));
#6032=DIRECTION('center_axis',(0.,1.,0.));
#6033=DIRECTION('ref_axis',(1.,0.,0.));
#6034=DIRECTION('center_axis',(0.,1.,0.));
#6035=DIRECTION('ref_axis',(1.,0.,0.));
#6036=DIRECTION('',(0.,1.,0.));
#6037=DIRECTION('center_axis',(0.,-1.,0.));
#6038=DIRECTION('ref_axis',(1.,0.,0.));
#6039=DIRECTION('center_axis',(0.,1.,0.));
#6040=DIRECTION('ref_axis',(1.,0.,0.));
#6041=DIRECTION('center_axis',(0.,1.,0.));
#6042=DIRECTION('ref_axis',(-1.,0.,0.));
#6043=DIRECTION('',(-1.,0.,0.));
#6044=DIRECTION('',(0.,0.,1.));
#6045=DIRECTION('',(-1.,0.,0.));
#6046=DIRECTION('',(0.,0.,1.));
#6047=DIRECTION('center_axis',(1.,0.,0.));
#6048=DIRECTION('ref_axis',(0.,1.,0.));
#6049=DIRECTION('',(0.,1.,0.));
#6050=DIRECTION('',(0.,1.,0.));
#6051=DIRECTION('',(0.,0.,1.));
#6052=DIRECTION('center_axis',(0.,-1.,0.));
#6053=DIRECTION('ref_axis',(1.,0.,0.));
#6054=DIRECTION('',(1.,0.,0.));
#6055=DIRECTION('',(1.,0.,0.));
#6056=DIRECTION('',(0.,0.,1.));
#6057=DIRECTION('center_axis',(-1.,0.,0.));
#6058=DIRECTION('ref_axis',(0.,-1.,0.));
#6059=DIRECTION('',(0.,-1.,0.));
#6060=DIRECTION('',(0.,-1.,0.));
#6061=DIRECTION('center_axis',(0.,0.,1.));
#6062=DIRECTION('ref_axis',(1.,0.,0.));
#6063=DIRECTION('center_axis',(0.,0.,1.));
#6064=DIRECTION('ref_axis',(1.,0.,0.));
#7498=CARTESIAN_POINT('',(0.,0.,0.));
#7499=CARTESIAN_POINT('Origin',(-1.2,0.6,1.9));
#7500=CARTESIAN_POINT('',(-1.41,0.6,2.));
#7501=CARTESIAN_POINT('Origin',(-1.2,0.6,2.));
#7502=CARTESIAN_POINT('',(-1.41,0.6,3.1));
#7503=CARTESIAN_POINT('',(-1.41,0.6,1.9));
#7504=CARTESIAN_POINT('Origin',(-1.2,0.6,3.1));
#7505=CARTESIAN_POINT('Origin',(-1.2,0.6,3.1));
#7506=CARTESIAN_POINT('Origin',(1.2,0.6,1.9));
#7507=CARTESIAN_POINT('',(0.99,0.6,2.));
#7508=CARTESIAN_POINT('Origin',(1.2,0.6,2.));
#7509=CARTESIAN_POINT('',(0.99,0.6,3.1));
#7510=CARTESIAN_POINT('',(0.99,0.6,1.9));
#7511=CARTESIAN_POINT('Origin',(1.2,0.6,3.1));
#7512=CARTESIAN_POINT('Origin',(1.2,0.6,3.1));
#7513=CARTESIAN_POINT('Origin',(0.,0.7,5.4));
#7514=CARTESIAN_POINT('',(0.173205080756888,0.7,5.3));
#7515=CARTESIAN_POINT('',(-0.173205080756888,0.7,5.3));
#7516=CARTESIAN_POINT('',(0.,0.7,5.3));
#7517=CARTESIAN_POINT('Origin',(0.,0.7,5.4));
#7518=CARTESIAN_POINT('Origin',(0.,0.7,5.4));
#7519=CARTESIAN_POINT('',(0.173205080756888,0.7,5.5));
#7520=CARTESIAN_POINT('',(0.173205080756888,0.7,5.3));
#7521=CARTESIAN_POINT('Origin',(0.,0.7,5.4));
#7522=CARTESIAN_POINT('Origin',(0.,0.7,5.4));
#7523=CARTESIAN_POINT('',(0.2,0.8,5.4));
#7524=CARTESIAN_POINT('Origin',(0.,0.8,5.4));
#7525=CARTESIAN_POINT('Origin',(0.,0.8,5.4));
#7526=CARTESIAN_POINT('Origin',(0.,0.7,5.4));
#7527=CARTESIAN_POINT('',(-0.173205080756888,0.9,5.3));
#7528=CARTESIAN_POINT('',(-0.173205080756888,0.7,5.3));
#7529=CARTESIAN_POINT('',(0.173205080756888,0.9,5.3));
#7530=CARTESIAN_POINT('',(0.173205080756888,0.7,5.3));
#7531=CARTESIAN_POINT('Origin',(0.,0.8,5.4));
#7532=CARTESIAN_POINT('',(-0.2,0.8,5.4));
#7533=CARTESIAN_POINT('Origin',(0.,0.8,5.4));
#7534=CARTESIAN_POINT('',(-0.2,1.2,5.4));
#7535=CARTESIAN_POINT('',(-0.2,0.7,5.4));
#7536=CARTESIAN_POINT('',(-0.181811868577262,1.2,5.48333333333333));
#7537=CARTESIAN_POINT('Origin',(0.,1.2,5.4));
#7538=CARTESIAN_POINT('',(-0.181811868577262,1.5,5.48333333333333));
#7539=CARTESIAN_POINT('',(-0.181811868577262,0.7,5.48333333333333));
#7540=CARTESIAN_POINT('',(0.181811868577262,1.5,5.48333333333333));
#7541=CARTESIAN_POINT('Origin',(0.,1.5,5.4));
#7542=CARTESIAN_POINT('',(0.181811868577262,1.2,5.48333333333333));
#7543=CARTESIAN_POINT('',(0.181811868577262,0.7,5.48333333333333));
#7544=CARTESIAN_POINT('Origin',(0.,1.2,5.4));
#7545=CARTESIAN_POINT('Origin',(0.,0.8,5.4));
#7546=CARTESIAN_POINT('Origin',(0.,0.7,5.4));
#7547=CARTESIAN_POINT('',(-0.173205080756888,0.7,5.5));
#7548=CARTESIAN_POINT('Origin',(0.,0.8,5.4));
#7549=CARTESIAN_POINT('Origin',(0.,0.7,5.4));
#7550=CARTESIAN_POINT('Origin',(0.,0.8,5.4));
#7551=CARTESIAN_POINT('Origin',(0.,1.5,5.4));
#7552=CARTESIAN_POINT('Origin',(0.,1.5,4.5));
#7553=CARTESIAN_POINT('Origin',(0.,0.7,5.4));
#7554=CARTESIAN_POINT('',(-0.173205080756888,0.7,5.3));
#7555=CARTESIAN_POINT('Origin',(0.,0.8,5.3));
#7556=CARTESIAN_POINT('Origin',(0.,0.8,5.3));
#7557=CARTESIAN_POINT('Origin',(0.,0.8,5.3));
#7558=CARTESIAN_POINT('Origin',(0.,0.8,5.3));
#7559=CARTESIAN_POINT('Origin',(0.,0.8,5.3));
#7560=CARTESIAN_POINT('Origin',(0.,0.8,5.3));
#7561=CARTESIAN_POINT('',(-0.2,0.8,5.8));
#7562=CARTESIAN_POINT('',(-0.2,0.8,5.3));
#7563=CARTESIAN_POINT('Origin',(0.,0.8,5.8));
#7564=CARTESIAN_POINT('Origin',(0.,0.8,5.3));
#7565=CARTESIAN_POINT('Origin',(0.,0.8,5.3));
#7566=CARTESIAN_POINT('Origin',(0.,1.2,4.5));
#7567=CARTESIAN_POINT('',(-1.,1.2,4.5));
#7568=CARTESIAN_POINT('Origin',(0.,1.2,4.5));
#7569=CARTESIAN_POINT('',(-1.,1.7,4.5));
#7570=CARTESIAN_POINT('',(-1.,1.2,4.5));
#7571=CARTESIAN_POINT('Origin',(0.,1.7,4.5));
#7572=CARTESIAN_POINT('Origin',(0.,1.2,4.5));
#7573=CARTESIAN_POINT('Origin',(0.,0.8,5.3));
#7574=CARTESIAN_POINT('Origin',(0.,0.8,5.8));
#7575=CARTESIAN_POINT('',(-0.685,0.8,5.8));
#7576=CARTESIAN_POINT('Origin',(0.,0.8,5.8));
#7577=CARTESIAN_POINT('',(-0.685,0.8,7.));
#7578=CARTESIAN_POINT('',(-0.685,0.8,5.8));
#7579=CARTESIAN_POINT('Origin',(0.,0.8,7.));
#7580=CARTESIAN_POINT('Origin',(0.,0.8,5.8));
#7581=CARTESIAN_POINT('Origin',(2.,-0.1,2.5));
#7582=CARTESIAN_POINT('',(1.725,0.,2.5));
#7583=CARTESIAN_POINT('Origin',(2.,0.,2.5));
#7584=CARTESIAN_POINT('',(1.725,1.7,2.5));
#7585=CARTESIAN_POINT('',(1.725,-0.1,2.5));
#7586=CARTESIAN_POINT('Origin',(2.,1.7,2.5));
#7587=CARTESIAN_POINT('Origin',(-2.,-0.1,6.5));
#7588=CARTESIAN_POINT('',(-2.275,0.,6.5));
#7589=CARTESIAN_POINT('Origin',(-2.,0.,6.5));
#7590=CARTESIAN_POINT('',(-2.275,1.7,6.5));
#7591=CARTESIAN_POINT('',(-2.275,-0.1,6.5));
#7592=CARTESIAN_POINT('Origin',(-2.,1.7,6.5));
#7593=CARTESIAN_POINT('Origin',(-2.,-0.1,2.5));
#7594=CARTESIAN_POINT('',(-2.275,0.,2.5));
#7595=CARTESIAN_POINT('Origin',(-2.,0.,2.5));
#7596=CARTESIAN_POINT('',(-2.275,1.7,2.5));
#7597=CARTESIAN_POINT('',(-2.275,-0.1,2.5));
#7598=CARTESIAN_POINT('Origin',(-2.,1.7,2.5));
#7599=CARTESIAN_POINT('Origin',(2.,-0.1,6.5));
#7600=CARTESIAN_POINT('',(1.725,0.,6.5));
#7601=CARTESIAN_POINT('Origin',(2.,0.,6.5));
#7602=CARTESIAN_POINT('',(1.725,1.7,6.5));
#7603=CARTESIAN_POINT('',(1.725,-0.1,6.5));
#7604=CARTESIAN_POINT('Origin',(2.,1.7,6.5));
#7605=CARTESIAN_POINT('Origin',(0.,-0.1,4.5));
#7606=CARTESIAN_POINT('',(-0.6,0.,4.5));
#7607=CARTESIAN_POINT('Origin',(0.,0.,4.5));
#7608=CARTESIAN_POINT('',(-0.6,1.2,4.5));
#7609=CARTESIAN_POINT('',(-0.6,-0.1,4.5));
#7610=CARTESIAN_POINT('Origin',(0.,1.2,4.5));
#7611=CARTESIAN_POINT('Origin',(0.,1.2,4.5));
#7612=CARTESIAN_POINT('Origin',(2.5,1.7,2.));
#7613=CARTESIAN_POINT('',(2.5,1.7,2.));
#7614=CARTESIAN_POINT('',(-2.5,1.7,2.));
#7615=CARTESIAN_POINT('',(2.5,1.7,2.));
#7616=CARTESIAN_POINT('',(-2.5,1.7,7.));
#7617=CARTESIAN_POINT('',(-2.5,1.7,2.));
#7618=CARTESIAN_POINT('',(2.5,1.7,7.));
#7619=CARTESIAN_POINT('',(2.5,1.7,7.));
#7620=CARTESIAN_POINT('',(2.5,1.7,2.));
#7621=CARTESIAN_POINT('Origin',(2.5,0.,2.));
#7622=CARTESIAN_POINT('',(2.5,0.,2.));
#7623=CARTESIAN_POINT('',(2.5,0.,2.));
#7624=CARTESIAN_POINT('',(2.5,0.,7.));
#7625=CARTESIAN_POINT('',(2.5,0.,7.));
#7626=CARTESIAN_POINT('',(2.5,0.,2.));
#7627=CARTESIAN_POINT('Origin',(-2.5,0.,2.));
#7628=CARTESIAN_POINT('',(-2.5,0.,2.));
#7629=CARTESIAN_POINT('',(-2.5,0.,2.));
#7630=CARTESIAN_POINT('',(-2.5,0.,7.));
#7631=CARTESIAN_POINT('',(-2.5,0.,7.));
#7632=CARTESIAN_POINT('',(-2.5,0.,2.));
#7633=CARTESIAN_POINT('Origin',(-2.5,1.7,2.));
#7634=CARTESIAN_POINT('',(-2.5,1.7,2.));
#7635=CARTESIAN_POINT('',(-2.5,1.7,7.));
#7636=CARTESIAN_POINT('Origin',(0.,0.85,7.));
#7637=CARTESIAN_POINT('Origin',(0.,0.85,2.));
#9039=UNCERTAINTY_MEASURE_WITH_UNIT(LENGTH_MEASURE(0.001),#9103,
'DISTANCE_ACCURACY_VALUE',
'Maximum model space distance between geometric entities at asserted c
onnectivities');
#9069=UNCERTAINTY_MEASURE_WITH_UNIT(LENGTH_MEASURE(0.001),#9103,
'DISTANCE_ACCURACY_VALUE',
'Maximum model space distance between geometric entities at asserted c
onnectivities');
#9072=(
GEOMETRIC_REPRESENTATION_CONTEXT(3)
GLOBAL_UNCERTAINTY_ASSIGNED_CONTEXT((#9039))
GLOBAL_UNIT_ASSIGNED_CONTEXT((#9103,#9105,#9106))
REPRESENTATION_CONTEXT('','3D')
);
#9102=(
GEOMETRIC_REPRESENTATION_CONTEXT(3)
GLOBAL_UNCERTAINTY_ASSIGNED_CONTEXT((#9069))
GLOBAL_UNIT_ASSIGNED_CONTEXT((#9103,#9105,#9106))
REPRESENTATION_CONTEXT('','3D')
);
#9103=(
LENGTH_UNIT()
NAMED_UNIT(*)
SI_UNIT(.CENTI.,.METRE.)
);
#9105=(
NAMED_UNIT(*)
PLANE_ANGLE_UNIT()
SI_UNIT($,.RADIAN.)
);
#9106=(
NAMED_UNIT(*)
SI_UNIT($,.STERADIAN.)
SOLID_ANGLE_UNIT()
);
#9109=SHAPE_DEFINITION_REPRESENTATION(#9141,#9229);
#9141=PRODUCT_DEFINITION_SHAPE('',$,#9262);
#9229=SHAPE_REPRESENTATION('',(#5265),#9072);
#9259=PRODUCT_DEFINITION_CONTEXT('part definition',#9357,'design');
#9262=PRODUCT_DEFINITION('Front cylinder cap','Front cylinder cap',#9294,
#9259);
#9294=PRODUCT_DEFINITION_FORMATION('',$,#9361);
#9357=APPLICATION_CONTEXT(
'Core Data for Automotive Mechanical Design Process');
#9358=PRODUCT_CONTEXT('part definition',#9357,'mechanical');
#9361=PRODUCT('Front cylinder cap','Front cylinder cap',
'Front cylinder cap',(#9358));
#9440=COLOUR_RGB('Light Blue',0.38,0.62,0.78);
#9441=FILL_AREA_STYLE_COLOUR('',#9440);
#9442=FILL_AREA_STYLE('',(#9441));
#9443=SURFACE_STYLE_FILL_AREA(#9442);
#9444=SURFACE_SIDE_STYLE('',(#9443));
#9445=SURFACE_STYLE_USAGE(.BOTH.,#9444);
#9446=PRESENTATION_STYLE_ASSIGNMENT((#9445));
ENDSEC;
END-ISO-10303-21;
